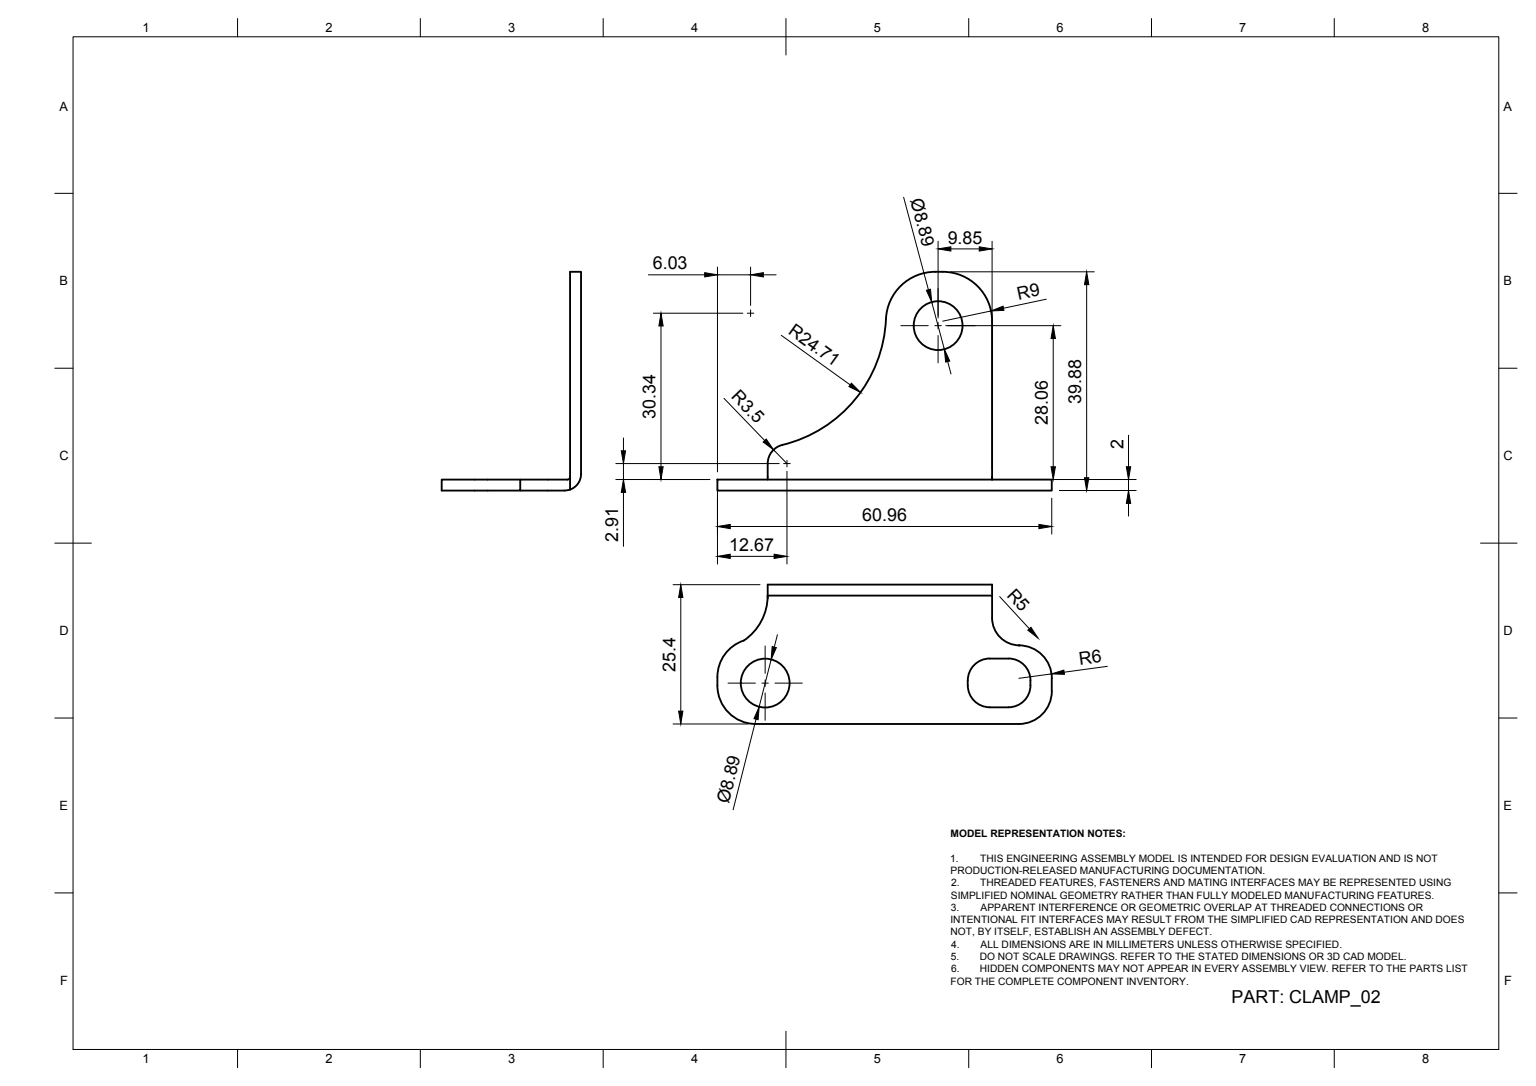
ISO-10303-21;
HEADER;
/* Generated by software containing ST-Developer
 * from STEP Tools, Inc. (www.steptools.com) 
 */

FILE_DESCRIPTION(
/* description */ (''),
/* implementation_level */ '2;1');

FILE_NAME(
/* name */ 'Clamp_02.step',
/* time_stamp */ '2026-10-04T16:49:01-07:00',
/* author */ (''),
/* organization */ (''),
/* preprocessor_version */ 'ST-DEVELOPER v20.2',
/* originating_system */ 'Autodesk Translation Framework v15.15.0.0',
/* authorisation */ '');

FILE_SCHEMA (('AUTOMOTIVE_DESIGN { 1 0 10303 214 3 1 1 }'));
ENDSEC;

DATA;
#10=MECHANICAL_DESIGN_GEOMETRIC_PRESENTATION_REPRESENTATION('',(#86),#51553);
#70=SHAPE_REPRESENTATION_RELATIONSHIP('SRR','None',#51591,#78);
#78=ADVANCED_BREP_SHAPE_REPRESENTATION('',(#95),#51551);
#86=STYLED_ITEM('',(#51634),#95);
#95=MANIFOLD_SOLID_BREP('Body1',#4265);
#110=FACE_BOUND('',#538,.T.);
#111=FACE_BOUND('',#541,.T.);
#112=FACE_BOUND('',#570,.T.);
#113=FACE_BOUND('',#571,.T.);
#114=FACE_BOUND('',#573,.T.);
#115=FACE_BOUND('',#574,.T.);
#159=PLANE('',#4564);
#160=PLANE('',#4566);
#161=PLANE('',#4572);
#162=PLANE('',#4573);
#163=PLANE('',#4584);
#164=PLANE('',#4587);
#165=PLANE('',#4591);
#166=PLANE('',#4595);
#167=PLANE('',#4599);
#168=PLANE('',#4603);
#169=PLANE('',#4616);
#170=PLANE('',#4620);
#171=PLANE('',#4624);
#172=PLANE('',#4628);
#173=PLANE('',#4629);
#174=PLANE('',#4630);
#328=FACE_OUTER_BOUND('',#535,.T.);
#329=FACE_OUTER_BOUND('',#536,.T.);
#330=FACE_OUTER_BOUND('',#537,.T.);
#331=FACE_OUTER_BOUND('',#539,.T.);
#332=FACE_OUTER_BOUND('',#540,.T.);
#333=FACE_OUTER_BOUND('',#542,.T.);
#334=FACE_OUTER_BOUND('',#543,.T.);
#335=FACE_OUTER_BOUND('',#544,.T.);
#336=FACE_OUTER_BOUND('',#545,.T.);
#337=FACE_OUTER_BOUND('',#546,.T.);
#338=FACE_OUTER_BOUND('',#547,.T.);
#339=FACE_OUTER_BOUND('',#548,.T.);
#340=FACE_OUTER_BOUND('',#549,.T.);
#341=FACE_OUTER_BOUND('',#550,.T.);
#342=FACE_OUTER_BOUND('',#551,.T.);
#343=FACE_OUTER_BOUND('',#552,.T.);
#344=FACE_OUTER_BOUND('',#553,.T.);
#345=FACE_OUTER_BOUND('',#554,.T.);
#346=FACE_OUTER_BOUND('',#555,.T.);
#347=FACE_OUTER_BOUND('',#556,.T.);
#348=FACE_OUTER_BOUND('',#557,.T.);
#349=FACE_OUTER_BOUND('',#558,.T.);
#350=FACE_OUTER_BOUND('',#559,.T.);
#351=FACE_OUTER_BOUND('',#560,.T.);
#352=FACE_OUTER_BOUND('',#561,.T.);
#353=FACE_OUTER_BOUND('',#562,.T.);
#354=FACE_OUTER_BOUND('',#563,.T.);
#355=FACE_OUTER_BOUND('',#564,.T.);
#356=FACE_OUTER_BOUND('',#565,.T.);
#357=FACE_OUTER_BOUND('',#566,.T.);
#358=FACE_OUTER_BOUND('',#567,.T.);
#359=FACE_OUTER_BOUND('',#568,.T.);
#360=FACE_OUTER_BOUND('',#569,.T.);
#361=FACE_OUTER_BOUND('',#572,.T.);
#535=EDGE_LOOP('',(#3703,#3704,#3705,#3706,#3707,#3708,#3709));
#536=EDGE_LOOP('',(#3710,#3711,#3712,#3713,#3714,#3715));
#537=EDGE_LOOP('',(#3716,#3717,#3718,#3719,#3720,#3721,#3722,#3723,#3724,
#3725));
#538=EDGE_LOOP('',(#3726));
#539=EDGE_LOOP('',(#3727,#3728,#3729,#3730));
#540=EDGE_LOOP('',(#3731,#3732,#3733,#3734,#3735,#3736,#3737,#3738));
#541=EDGE_LOOP('',(#3739));
#542=EDGE_LOOP('',(#3740,#3741,#3742,#3743));
#543=EDGE_LOOP('',(#3744,#3745,#3746,#3747));
#544=EDGE_LOOP('',(#3748,#3749,#3750,#3751));
#545=EDGE_LOOP('',(#3752,#3753,#3754,#3755));
#546=EDGE_LOOP('',(#3756,#3757,#3758,#3759));
#547=EDGE_LOOP('',(#3760,#3761,#3762,#3763));
#548=EDGE_LOOP('',(#3764,#3765,#3766,#3767));
#549=EDGE_LOOP('',(#3768,#3769,#3770,#3771,#3772,#3773,#3774));
#550=EDGE_LOOP('',(#3775,#3776,#3777,#3778));
#551=EDGE_LOOP('',(#3779,#3780,#3781,#3782));
#552=EDGE_LOOP('',(#3783,#3784,#3785,#3786));
#553=EDGE_LOOP('',(#3787,#3788,#3789,#3790));
#554=EDGE_LOOP('',(#3791,#3792,#3793,#3794));
#555=EDGE_LOOP('',(#3795,#3796,#3797,#3798));
#556=EDGE_LOOP('',(#3799,#3800,#3801,#3802));
#557=EDGE_LOOP('',(#3803,#3804,#3805,#3806));
#558=EDGE_LOOP('',(#3807,#3808,#3809,#3810));
#559=EDGE_LOOP('',(#3811,#3812,#3813,#3814));
#560=EDGE_LOOP('',(#3815,#3816,#3817,#3818,#3819));
#561=EDGE_LOOP('',(#3820,#3821,#3822,#3823));
#562=EDGE_LOOP('',(#3824,#3825,#3826,#3827));
#563=EDGE_LOOP('',(#3828,#3829,#3830,#3831));
#564=EDGE_LOOP('',(#3832,#3833,#3834,#3835));
#565=EDGE_LOOP('',(#3836,#3837,#3838,#3839));
#566=EDGE_LOOP('',(#3840,#3841,#3842,#3843));
#567=EDGE_LOOP('',(#3844,#3845,#3846,#3847));
#568=EDGE_LOOP('',(#3848,#3849,#3850,#3851));
#569=EDGE_LOOP('',(#3852,#3853,#3854,#3855,#3856,#3857,#3858,#3859,#3860,
#3861,#3862,#3863,#3864));
#570=EDGE_LOOP('',(#3865,#3866,#3867,#3868,#3869,#3870,#3871,#3872));
#571=EDGE_LOOP('',(#3873));
#572=EDGE_LOOP('',(#3874,#3875,#3876,#3877,#3878,#3879,#3880,#3881,#3882,
#3883,#3884,#3885));
#573=EDGE_LOOP('',(#3886,#3887,#3888,#3889,#3890,#3891,#3892,#3893));
#574=EDGE_LOOP('',(#3894));
#657=CIRCLE('',#4561,3.);
#658=CIRCLE('',#4562,3.);
#659=CIRCLE('',#4563,3.);
#660=CIRCLE('',#4565,0.5);
#661=CIRCLE('',#4567,9.);
#662=CIRCLE('',#4568,9.);
#663=CIRCLE('',#4569,24.7141941620437);
#664=CIRCLE('',#4570,3.5);
#665=CIRCLE('',#4571,4.445);
#666=CIRCLE('',#4574,3.5);
#667=CIRCLE('',#4575,24.7141941620437);
#668=CIRCLE('',#4576,9.);
#669=CIRCLE('',#4577,9.);
#670=CIRCLE('',#4578,4.445);
#671=CIRCLE('',#4580,0.5);
#672=CIRCLE('',#4589,4.445);
#673=CIRCLE('',#4590,4.445);
#674=CIRCLE('',#4593,3.99999999999999);
#675=CIRCLE('',#4594,3.99999999999999);
#676=CIRCLE('',#4597,4.00000000000001);
#677=CIRCLE('',#4598,4.00000000000001);
#678=CIRCLE('',#4601,4.00000000000001);
#679=CIRCLE('',#4602,4.00000000000001);
#680=CIRCLE('',#4605,4.00000000000001);
#681=CIRCLE('',#4606,4.00000000000001);
#682=CIRCLE('',#4608,6.99999999999999);
#683=CIRCLE('',#4609,6.99999999999999);
#684=CIRCLE('',#4611,9.9094315895918);
#685=CIRCLE('',#4612,9.9094315895918);
#686=CIRCLE('',#4614,5.);
#687=CIRCLE('',#4615,5.);
#688=CIRCLE('',#4618,5.99999999999999);
#689=CIRCLE('',#4619,5.99999999999999);
#690=CIRCLE('',#4622,5.99999999999999);
#691=CIRCLE('',#4623,5.99999999999999);
#692=CIRCLE('',#4626,7.);
#693=CIRCLE('',#4627,7.);
#872=LINE('',#51257,#1100);
#873=LINE('',#51261,#1101);
#874=LINE('',#51265,#1102);
#875=LINE('',#51272,#1103);
#876=LINE('',#51276,#1104);
#877=LINE('',#51278,#1105);
#878=LINE('',#51279,#1106);
#879=LINE('',#51282,#1107);
#880=LINE('',#51286,#1108);
#881=LINE('',#51294,#1109);
#882=LINE('',#51295,#1110);
#883=LINE('',#51300,#1111);
#884=LINE('',#51301,#1112);
#885=LINE('',#51304,#1113);
#886=LINE('',#51312,#1114);
#887=LINE('',#51319,#1115);
#888=LINE('',#51321,#1116);
#889=LINE('',#51322,#1117);
#890=LINE('',#51324,#1118);
#891=LINE('',#51326,#1119);
#892=LINE('',#51328,#1120);
#893=LINE('',#51331,#1121);
#894=LINE('',#51334,#1122);
#895=LINE('',#51335,#1123);
#896=LINE('',#51340,#1124);
#897=LINE('',#51345,#1125);
#898=LINE('',#51347,#1126);
#899=LINE('',#51349,#1127);
#900=LINE('',#51350,#1128);
#901=LINE('',#51356,#1129);
#902=LINE('',#51359,#1130);
#903=LINE('',#51361,#1131);
#904=LINE('',#51362,#1132);
#905=LINE('',#51368,#1133);
#906=LINE('',#51371,#1134);
#907=LINE('',#51373,#1135);
#908=LINE('',#51374,#1136);
#909=LINE('',#51380,#1137);
#910=LINE('',#51383,#1138);
#911=LINE('',#51385,#1139);
#912=LINE('',#51386,#1140);
#913=LINE('',#51395,#1141);
#914=LINE('',#51398,#1142);
#915=LINE('',#51407,#1143);
#916=LINE('',#51410,#1144);
#917=LINE('',#51412,#1145);
#918=LINE('',#51413,#1146);
#919=LINE('',#51419,#1147);
#920=LINE('',#51422,#1148);
#921=LINE('',#51424,#1149);
#922=LINE('',#51425,#1150);
#923=LINE('',#51431,#1151);
#924=LINE('',#51434,#1152);
#925=LINE('',#51436,#1153);
#926=LINE('',#51437,#1154);
#927=LINE('',#51443,#1155);
#928=LINE('',#51445,#1156);
#929=LINE('',#51446,#1157);
#1100=VECTOR('',#5242,10.);
#1101=VECTOR('',#5245,10.);
#1102=VECTOR('',#5248,10.);
#1103=VECTOR('',#5251,10.);
#1104=VECTOR('',#5254,10.);
#1105=VECTOR('',#5255,10.);
#1106=VECTOR('',#5256,10.);
#1107=VECTOR('',#5259,10.);
#1108=VECTOR('',#5262,10.);
#1109=VECTOR('',#5269,10.);
#1110=VECTOR('',#5270,10.);
#1111=VECTOR('',#5275,10.);
#1112=VECTOR('',#5276,10.);
#1113=VECTOR('',#5279,10.);
#1114=VECTOR('',#5286,10.);
#1115=VECTOR('',#5295,10.);
#1116=VECTOR('',#5298,10.);
#1117=VECTOR('',#5299,10.);
#1118=VECTOR('',#5302,9.);
#1119=VECTOR('',#5305,10.);
#1120=VECTOR('',#5308,9.);
#1121=VECTOR('',#5313,4.445);
#1122=VECTOR('',#5316,10.);
#1123=VECTOR('',#5317,10.);
#1124=VECTOR('',#5322,4.445);
#1125=VECTOR('',#5327,10.);
#1126=VECTOR('',#5328,10.);
#1127=VECTOR('',#5329,10.);
#1128=VECTOR('',#5330,10.);
#1129=VECTOR('',#5337,10.);
#1130=VECTOR('',#5340,10.);
#1131=VECTOR('',#5341,10.);
#1132=VECTOR('',#5342,10.);
#1133=VECTOR('',#5349,10.);
#1134=VECTOR('',#5352,10.);
#1135=VECTOR('',#5353,10.);
#1136=VECTOR('',#5354,10.);
#1137=VECTOR('',#5361,10.);
#1138=VECTOR('',#5364,10.);
#1139=VECTOR('',#5365,10.);
#1140=VECTOR('',#5366,10.);
#1141=VECTOR('',#5377,10.);
#1142=VECTOR('',#5380,10.);
#1143=VECTOR('',#5393,10.);
#1144=VECTOR('',#5396,10.);
#1145=VECTOR('',#5397,10.);
#1146=VECTOR('',#5398,10.);
#1147=VECTOR('',#5405,10.);
#1148=VECTOR('',#5408,10.);
#1149=VECTOR('',#5409,10.);
#1150=VECTOR('',#5410,10.);
#1151=VECTOR('',#5417,10.);
#1152=VECTOR('',#5420,10.);
#1153=VECTOR('',#5421,10.);
#1154=VECTOR('',#5422,10.);
#1155=VECTOR('',#5429,10.);
#1156=VECTOR('',#5432,10.);
#1157=VECTOR('',#5433,10.);
#1479=B_SPLINE_CURVE_WITH_KNOTS('',3,(#51266,#51267,#51268,#51269),
 .UNSPECIFIED.,.F.,.F.,(4,4),(-0.453207372117249,-0.354837975954888),
 .UNSPECIFIED.);
#1884=VERTEX_POINT('',#51253);
#1885=VERTEX_POINT('',#51254);
#1886=VERTEX_POINT('',#51256);
#1887=VERTEX_POINT('',#51258);
#1888=VERTEX_POINT('',#51260);
#1889=VERTEX_POINT('',#51262);
#1890=VERTEX_POINT('',#51264);
#1891=VERTEX_POINT('',#51271);
#1892=VERTEX_POINT('',#51273);
#1893=VERTEX_POINT('',#51275);
#1894=VERTEX_POINT('',#51277);
#1895=VERTEX_POINT('',#51281);
#1896=VERTEX_POINT('',#51283);
#1897=VERTEX_POINT('',#51285);
#1898=VERTEX_POINT('',#51287);
#1899=VERTEX_POINT('',#51289);
#1900=VERTEX_POINT('',#51291);
#1901=VERTEX_POINT('',#51293);
#1902=VERTEX_POINT('',#51296);
#1903=VERTEX_POINT('',#51299);
#1904=VERTEX_POINT('',#51303);
#1905=VERTEX_POINT('',#51305);
#1906=VERTEX_POINT('',#51307);
#1907=VERTEX_POINT('',#51309);
#1908=VERTEX_POINT('',#51311);
#1909=VERTEX_POINT('',#51314);
#1910=VERTEX_POINT('',#51317);
#1911=VERTEX_POINT('',#51333);
#1912=VERTEX_POINT('',#51337);
#1913=VERTEX_POINT('',#51339);
#1914=VERTEX_POINT('',#51343);
#1915=VERTEX_POINT('',#51344);
#1916=VERTEX_POINT('',#51346);
#1917=VERTEX_POINT('',#51348);
#1918=VERTEX_POINT('',#51352);
#1919=VERTEX_POINT('',#51354);
#1920=VERTEX_POINT('',#51358);
#1921=VERTEX_POINT('',#51360);
#1922=VERTEX_POINT('',#51364);
#1923=VERTEX_POINT('',#51366);
#1924=VERTEX_POINT('',#51370);
#1925=VERTEX_POINT('',#51372);
#1926=VERTEX_POINT('',#51376);
#1927=VERTEX_POINT('',#51378);
#1928=VERTEX_POINT('',#51382);
#1929=VERTEX_POINT('',#51384);
#1930=VERTEX_POINT('',#51391);
#1931=VERTEX_POINT('',#51392);
#1932=VERTEX_POINT('',#51394);
#1933=VERTEX_POINT('',#51396);
#1934=VERTEX_POINT('',#51403);
#1935=VERTEX_POINT('',#51405);
#1936=VERTEX_POINT('',#51409);
#1937=VERTEX_POINT('',#51411);
#1938=VERTEX_POINT('',#51415);
#1939=VERTEX_POINT('',#51417);
#1940=VERTEX_POINT('',#51421);
#1941=VERTEX_POINT('',#51423);
#1942=VERTEX_POINT('',#51427);
#1943=VERTEX_POINT('',#51429);
#1944=VERTEX_POINT('',#51433);
#1945=VERTEX_POINT('',#51435);
#1946=VERTEX_POINT('',#51439);
#1947=VERTEX_POINT('',#51441);
#2505=EDGE_CURVE('',#1884,#1885,#657,.T.);
#2506=EDGE_CURVE('',#1885,#1886,#872,.T.);
#2507=EDGE_CURVE('',#1886,#1887,#658,.T.);
#2508=EDGE_CURVE('',#1887,#1888,#873,.T.);
#2509=EDGE_CURVE('',#1888,#1889,#659,.T.);
#2510=EDGE_CURVE('',#1889,#1890,#874,.T.);
#2511=EDGE_CURVE('',#1890,#1884,#1479,.T.);
#2512=EDGE_CURVE('',#1888,#1891,#875,.T.);
#2513=EDGE_CURVE('',#1892,#1891,#660,.T.);
#2514=EDGE_CURVE('',#1893,#1892,#876,.T.);
#2515=EDGE_CURVE('',#1894,#1893,#877,.T.);
#2516=EDGE_CURVE('',#1894,#1889,#878,.T.);
#2517=EDGE_CURVE('',#1887,#1895,#879,.F.);
#2518=EDGE_CURVE('',#1896,#1895,#661,.T.);
#2519=EDGE_CURVE('',#1897,#1896,#880,.T.);
#2520=EDGE_CURVE('',#1898,#1897,#662,.T.);
#2521=EDGE_CURVE('',#1898,#1899,#663,.T.);
#2522=EDGE_CURVE('',#1900,#1899,#664,.T.);
#2523=EDGE_CURVE('',#1901,#1900,#881,.T.);
#2524=EDGE_CURVE('',#1891,#1901,#882,.T.);
#2525=EDGE_CURVE('',#1902,#1902,#665,.T.);
#2526=EDGE_CURVE('',#1886,#1903,#883,.T.);
#2527=EDGE_CURVE('',#1895,#1903,#884,.T.);
#2528=EDGE_CURVE('',#1885,#1904,#885,.F.);
#2529=EDGE_CURVE('',#1905,#1904,#666,.T.);
#2530=EDGE_CURVE('',#1905,#1906,#667,.T.);
#2531=EDGE_CURVE('',#1907,#1906,#668,.T.);
#2532=EDGE_CURVE('',#1908,#1907,#886,.T.);
#2533=EDGE_CURVE('',#1903,#1908,#669,.T.);
#2534=EDGE_CURVE('',#1909,#1909,#670,.T.);
#2535=EDGE_CURVE('',#1910,#1901,#671,.F.);
#2536=EDGE_CURVE('',#1910,#1892,#887,.T.);
#2537=EDGE_CURVE('',#1904,#1900,#888,.T.);
#2538=EDGE_CURVE('',#1899,#1905,#889,.T.);
#2539=EDGE_CURVE('',#1906,#1898,#890,.T.);
#2540=EDGE_CURVE('',#1908,#1896,#891,.T.);
#2541=EDGE_CURVE('',#1897,#1907,#892,.T.);
#2542=EDGE_CURVE('',#1902,#1909,#893,.T.);
#2543=EDGE_CURVE('',#1884,#1911,#894,.T.);
#2544=EDGE_CURVE('',#1910,#1911,#895,.T.);
#2545=EDGE_CURVE('',#1912,#1912,#672,.T.);
#2546=EDGE_CURVE('',#1912,#1913,#896,.T.);
#2547=EDGE_CURVE('',#1913,#1913,#673,.T.);
#2548=EDGE_CURVE('',#1914,#1915,#897,.T.);
#2549=EDGE_CURVE('',#1915,#1916,#898,.T.);
#2550=EDGE_CURVE('',#1917,#1916,#899,.T.);
#2551=EDGE_CURVE('',#1914,#1917,#900,.T.);
#2552=EDGE_CURVE('',#1918,#1914,#674,.T.);
#2553=EDGE_CURVE('',#1919,#1917,#675,.T.);
#2554=EDGE_CURVE('',#1918,#1919,#901,.T.);
#2555=EDGE_CURVE('',#1920,#1918,#902,.T.);
#2556=EDGE_CURVE('',#1921,#1919,#903,.T.);
#2557=EDGE_CURVE('',#1920,#1921,#904,.T.);
#2558=EDGE_CURVE('',#1922,#1920,#676,.T.);
#2559=EDGE_CURVE('',#1923,#1921,#677,.T.);
#2560=EDGE_CURVE('',#1922,#1923,#905,.T.);
#2561=EDGE_CURVE('',#1924,#1922,#906,.T.);
#2562=EDGE_CURVE('',#1925,#1923,#907,.T.);
#2563=EDGE_CURVE('',#1924,#1925,#908,.T.);
#2564=EDGE_CURVE('',#1926,#1924,#678,.T.);
#2565=EDGE_CURVE('',#1927,#1925,#679,.T.);
#2566=EDGE_CURVE('',#1926,#1927,#909,.T.);
#2567=EDGE_CURVE('',#1928,#1926,#910,.T.);
#2568=EDGE_CURVE('',#1929,#1927,#911,.T.);
#2569=EDGE_CURVE('',#1928,#1929,#912,.T.);
#2570=EDGE_CURVE('',#1915,#1928,#680,.T.);
#2571=EDGE_CURVE('',#1916,#1929,#681,.T.);
#2572=EDGE_CURVE('',#1930,#1931,#682,.T.);
#2573=EDGE_CURVE('',#1931,#1932,#913,.T.);
#2574=EDGE_CURVE('',#1933,#1932,#683,.T.);
#2575=EDGE_CURVE('',#1930,#1933,#914,.T.);
#2576=EDGE_CURVE('',#1930,#1890,#684,.T.);
#2577=EDGE_CURVE('',#1911,#1933,#685,.T.);
#2578=EDGE_CURVE('',#1894,#1934,#686,.T.);
#2579=EDGE_CURVE('',#1935,#1893,#687,.T.);
#2580=EDGE_CURVE('',#1934,#1935,#915,.T.);
#2581=EDGE_CURVE('',#1936,#1934,#916,.T.);
#2582=EDGE_CURVE('',#1937,#1935,#917,.T.);
#2583=EDGE_CURVE('',#1936,#1937,#918,.T.);
#2584=EDGE_CURVE('',#1938,#1936,#688,.T.);
#2585=EDGE_CURVE('',#1939,#1937,#689,.T.);
#2586=EDGE_CURVE('',#1938,#1939,#919,.T.);
#2587=EDGE_CURVE('',#1940,#1938,#920,.T.);
#2588=EDGE_CURVE('',#1941,#1939,#921,.T.);
#2589=EDGE_CURVE('',#1940,#1941,#922,.T.);
#2590=EDGE_CURVE('',#1942,#1940,#690,.T.);
#2591=EDGE_CURVE('',#1943,#1941,#691,.T.);
#2592=EDGE_CURVE('',#1942,#1943,#923,.T.);
#2593=EDGE_CURVE('',#1944,#1942,#924,.T.);
#2594=EDGE_CURVE('',#1945,#1943,#925,.T.);
#2595=EDGE_CURVE('',#1944,#1945,#926,.T.);
#2596=EDGE_CURVE('',#1946,#1944,#692,.T.);
#2597=EDGE_CURVE('',#1947,#1945,#693,.T.);
#2598=EDGE_CURVE('',#1946,#1947,#927,.T.);
#2599=EDGE_CURVE('',#1931,#1946,#928,.T.);
#2600=EDGE_CURVE('',#1932,#1947,#929,.T.);
#3703=ORIENTED_EDGE('',*,*,#2505,.T.);
#3704=ORIENTED_EDGE('',*,*,#2506,.T.);
#3705=ORIENTED_EDGE('',*,*,#2507,.T.);
#3706=ORIENTED_EDGE('',*,*,#2508,.T.);
#3707=ORIENTED_EDGE('',*,*,#2509,.T.);
#3708=ORIENTED_EDGE('',*,*,#2510,.T.);
#3709=ORIENTED_EDGE('',*,*,#2511,.T.);
#3710=ORIENTED_EDGE('',*,*,#2509,.F.);
#3711=ORIENTED_EDGE('',*,*,#2512,.T.);
#3712=ORIENTED_EDGE('',*,*,#2513,.F.);
#3713=ORIENTED_EDGE('',*,*,#2514,.F.);
#3714=ORIENTED_EDGE('',*,*,#2515,.F.);
#3715=ORIENTED_EDGE('',*,*,#2516,.T.);
#3716=ORIENTED_EDGE('',*,*,#2508,.F.);
#3717=ORIENTED_EDGE('',*,*,#2517,.T.);
#3718=ORIENTED_EDGE('',*,*,#2518,.F.);
#3719=ORIENTED_EDGE('',*,*,#2519,.F.);
#3720=ORIENTED_EDGE('',*,*,#2520,.F.);
#3721=ORIENTED_EDGE('',*,*,#2521,.T.);
#3722=ORIENTED_EDGE('',*,*,#2522,.F.);
#3723=ORIENTED_EDGE('',*,*,#2523,.F.);
#3724=ORIENTED_EDGE('',*,*,#2524,.F.);
#3725=ORIENTED_EDGE('',*,*,#2512,.F.);
#3726=ORIENTED_EDGE('',*,*,#2525,.T.);
#3727=ORIENTED_EDGE('',*,*,#2507,.F.);
#3728=ORIENTED_EDGE('',*,*,#2526,.T.);
#3729=ORIENTED_EDGE('',*,*,#2527,.F.);
#3730=ORIENTED_EDGE('',*,*,#2517,.F.);
#3731=ORIENTED_EDGE('',*,*,#2506,.F.);
#3732=ORIENTED_EDGE('',*,*,#2528,.T.);
#3733=ORIENTED_EDGE('',*,*,#2529,.F.);
#3734=ORIENTED_EDGE('',*,*,#2530,.T.);
#3735=ORIENTED_EDGE('',*,*,#2531,.F.);
#3736=ORIENTED_EDGE('',*,*,#2532,.F.);
#3737=ORIENTED_EDGE('',*,*,#2533,.F.);
#3738=ORIENTED_EDGE('',*,*,#2526,.F.);
#3739=ORIENTED_EDGE('',*,*,#2534,.T.);
#3740=ORIENTED_EDGE('',*,*,#2535,.F.);
#3741=ORIENTED_EDGE('',*,*,#2536,.T.);
#3742=ORIENTED_EDGE('',*,*,#2513,.T.);
#3743=ORIENTED_EDGE('',*,*,#2524,.T.);
#3744=ORIENTED_EDGE('',*,*,#2529,.T.);
#3745=ORIENTED_EDGE('',*,*,#2537,.T.);
#3746=ORIENTED_EDGE('',*,*,#2522,.T.);
#3747=ORIENTED_EDGE('',*,*,#2538,.T.);
#3748=ORIENTED_EDGE('',*,*,#2538,.F.);
#3749=ORIENTED_EDGE('',*,*,#2521,.F.);
#3750=ORIENTED_EDGE('',*,*,#2539,.F.);
#3751=ORIENTED_EDGE('',*,*,#2530,.F.);
#3752=ORIENTED_EDGE('',*,*,#2533,.T.);
#3753=ORIENTED_EDGE('',*,*,#2540,.T.);
#3754=ORIENTED_EDGE('',*,*,#2518,.T.);
#3755=ORIENTED_EDGE('',*,*,#2527,.T.);
#3756=ORIENTED_EDGE('',*,*,#2540,.F.);
#3757=ORIENTED_EDGE('',*,*,#2532,.T.);
#3758=ORIENTED_EDGE('',*,*,#2541,.F.);
#3759=ORIENTED_EDGE('',*,*,#2519,.T.);
#3760=ORIENTED_EDGE('',*,*,#2531,.T.);
#3761=ORIENTED_EDGE('',*,*,#2539,.T.);
#3762=ORIENTED_EDGE('',*,*,#2520,.T.);
#3763=ORIENTED_EDGE('',*,*,#2541,.T.);
#3764=ORIENTED_EDGE('',*,*,#2525,.F.);
#3765=ORIENTED_EDGE('',*,*,#2542,.T.);
#3766=ORIENTED_EDGE('',*,*,#2534,.F.);
#3767=ORIENTED_EDGE('',*,*,#2542,.F.);
#3768=ORIENTED_EDGE('',*,*,#2505,.F.);
#3769=ORIENTED_EDGE('',*,*,#2543,.T.);
#3770=ORIENTED_EDGE('',*,*,#2544,.F.);
#3771=ORIENTED_EDGE('',*,*,#2535,.T.);
#3772=ORIENTED_EDGE('',*,*,#2523,.T.);
#3773=ORIENTED_EDGE('',*,*,#2537,.F.);
#3774=ORIENTED_EDGE('',*,*,#2528,.F.);
#3775=ORIENTED_EDGE('',*,*,#2545,.T.);
#3776=ORIENTED_EDGE('',*,*,#2546,.T.);
#3777=ORIENTED_EDGE('',*,*,#2547,.F.);
#3778=ORIENTED_EDGE('',*,*,#2546,.F.);
#3779=ORIENTED_EDGE('',*,*,#2548,.T.);
#3780=ORIENTED_EDGE('',*,*,#2549,.T.);
#3781=ORIENTED_EDGE('',*,*,#2550,.F.);
#3782=ORIENTED_EDGE('',*,*,#2551,.F.);
#3783=ORIENTED_EDGE('',*,*,#2552,.T.);
#3784=ORIENTED_EDGE('',*,*,#2551,.T.);
#3785=ORIENTED_EDGE('',*,*,#2553,.F.);
#3786=ORIENTED_EDGE('',*,*,#2554,.F.);
#3787=ORIENTED_EDGE('',*,*,#2555,.T.);
#3788=ORIENTED_EDGE('',*,*,#2554,.T.);
#3789=ORIENTED_EDGE('',*,*,#2556,.F.);
#3790=ORIENTED_EDGE('',*,*,#2557,.F.);
#3791=ORIENTED_EDGE('',*,*,#2558,.T.);
#3792=ORIENTED_EDGE('',*,*,#2557,.T.);
#3793=ORIENTED_EDGE('',*,*,#2559,.F.);
#3794=ORIENTED_EDGE('',*,*,#2560,.F.);
#3795=ORIENTED_EDGE('',*,*,#2561,.T.);
#3796=ORIENTED_EDGE('',*,*,#2560,.T.);
#3797=ORIENTED_EDGE('',*,*,#2562,.F.);
#3798=ORIENTED_EDGE('',*,*,#2563,.F.);
#3799=ORIENTED_EDGE('',*,*,#2564,.T.);
#3800=ORIENTED_EDGE('',*,*,#2563,.T.);
#3801=ORIENTED_EDGE('',*,*,#2565,.F.);
#3802=ORIENTED_EDGE('',*,*,#2566,.F.);
#3803=ORIENTED_EDGE('',*,*,#2567,.T.);
#3804=ORIENTED_EDGE('',*,*,#2566,.T.);
#3805=ORIENTED_EDGE('',*,*,#2568,.F.);
#3806=ORIENTED_EDGE('',*,*,#2569,.F.);
#3807=ORIENTED_EDGE('',*,*,#2570,.T.);
#3808=ORIENTED_EDGE('',*,*,#2569,.T.);
#3809=ORIENTED_EDGE('',*,*,#2571,.F.);
#3810=ORIENTED_EDGE('',*,*,#2549,.F.);
#3811=ORIENTED_EDGE('',*,*,#2572,.T.);
#3812=ORIENTED_EDGE('',*,*,#2573,.T.);
#3813=ORIENTED_EDGE('',*,*,#2574,.F.);
#3814=ORIENTED_EDGE('',*,*,#2575,.F.);
#3815=ORIENTED_EDGE('',*,*,#2511,.F.);
#3816=ORIENTED_EDGE('',*,*,#2576,.F.);
#3817=ORIENTED_EDGE('',*,*,#2575,.T.);
#3818=ORIENTED_EDGE('',*,*,#2577,.F.);
#3819=ORIENTED_EDGE('',*,*,#2543,.F.);
#3820=ORIENTED_EDGE('',*,*,#2578,.F.);
#3821=ORIENTED_EDGE('',*,*,#2515,.T.);
#3822=ORIENTED_EDGE('',*,*,#2579,.F.);
#3823=ORIENTED_EDGE('',*,*,#2580,.F.);
#3824=ORIENTED_EDGE('',*,*,#2581,.T.);
#3825=ORIENTED_EDGE('',*,*,#2580,.T.);
#3826=ORIENTED_EDGE('',*,*,#2582,.F.);
#3827=ORIENTED_EDGE('',*,*,#2583,.F.);
#3828=ORIENTED_EDGE('',*,*,#2584,.T.);
#3829=ORIENTED_EDGE('',*,*,#2583,.T.);
#3830=ORIENTED_EDGE('',*,*,#2585,.F.);
#3831=ORIENTED_EDGE('',*,*,#2586,.F.);
#3832=ORIENTED_EDGE('',*,*,#2587,.T.);
#3833=ORIENTED_EDGE('',*,*,#2586,.T.);
#3834=ORIENTED_EDGE('',*,*,#2588,.F.);
#3835=ORIENTED_EDGE('',*,*,#2589,.F.);
#3836=ORIENTED_EDGE('',*,*,#2590,.T.);
#3837=ORIENTED_EDGE('',*,*,#2589,.T.);
#3838=ORIENTED_EDGE('',*,*,#2591,.F.);
#3839=ORIENTED_EDGE('',*,*,#2592,.F.);
#3840=ORIENTED_EDGE('',*,*,#2593,.T.);
#3841=ORIENTED_EDGE('',*,*,#2592,.T.);
#3842=ORIENTED_EDGE('',*,*,#2594,.F.);
#3843=ORIENTED_EDGE('',*,*,#2595,.F.);
#3844=ORIENTED_EDGE('',*,*,#2596,.T.);
#3845=ORIENTED_EDGE('',*,*,#2595,.T.);
#3846=ORIENTED_EDGE('',*,*,#2597,.F.);
#3847=ORIENTED_EDGE('',*,*,#2598,.F.);
#3848=ORIENTED_EDGE('',*,*,#2599,.T.);
#3849=ORIENTED_EDGE('',*,*,#2598,.T.);
#3850=ORIENTED_EDGE('',*,*,#2600,.F.);
#3851=ORIENTED_EDGE('',*,*,#2573,.F.);
#3852=ORIENTED_EDGE('',*,*,#2577,.T.);
#3853=ORIENTED_EDGE('',*,*,#2574,.T.);
#3854=ORIENTED_EDGE('',*,*,#2600,.T.);
#3855=ORIENTED_EDGE('',*,*,#2597,.T.);
#3856=ORIENTED_EDGE('',*,*,#2594,.T.);
#3857=ORIENTED_EDGE('',*,*,#2591,.T.);
#3858=ORIENTED_EDGE('',*,*,#2588,.T.);
#3859=ORIENTED_EDGE('',*,*,#2585,.T.);
#3860=ORIENTED_EDGE('',*,*,#2582,.T.);
#3861=ORIENTED_EDGE('',*,*,#2579,.T.);
#3862=ORIENTED_EDGE('',*,*,#2514,.T.);
#3863=ORIENTED_EDGE('',*,*,#2536,.F.);
#3864=ORIENTED_EDGE('',*,*,#2544,.T.);
#3865=ORIENTED_EDGE('',*,*,#2571,.T.);
#3866=ORIENTED_EDGE('',*,*,#2568,.T.);
#3867=ORIENTED_EDGE('',*,*,#2565,.T.);
#3868=ORIENTED_EDGE('',*,*,#2562,.T.);
#3869=ORIENTED_EDGE('',*,*,#2559,.T.);
#3870=ORIENTED_EDGE('',*,*,#2556,.T.);
#3871=ORIENTED_EDGE('',*,*,#2553,.T.);
#3872=ORIENTED_EDGE('',*,*,#2550,.T.);
#3873=ORIENTED_EDGE('',*,*,#2547,.T.);
#3874=ORIENTED_EDGE('',*,*,#2510,.F.);
#3875=ORIENTED_EDGE('',*,*,#2516,.F.);
#3876=ORIENTED_EDGE('',*,*,#2578,.T.);
#3877=ORIENTED_EDGE('',*,*,#2581,.F.);
#3878=ORIENTED_EDGE('',*,*,#2584,.F.);
#3879=ORIENTED_EDGE('',*,*,#2587,.F.);
#3880=ORIENTED_EDGE('',*,*,#2590,.F.);
#3881=ORIENTED_EDGE('',*,*,#2593,.F.);
#3882=ORIENTED_EDGE('',*,*,#2596,.F.);
#3883=ORIENTED_EDGE('',*,*,#2599,.F.);
#3884=ORIENTED_EDGE('',*,*,#2572,.F.);
#3885=ORIENTED_EDGE('',*,*,#2576,.T.);
#3886=ORIENTED_EDGE('',*,*,#2570,.F.);
#3887=ORIENTED_EDGE('',*,*,#2548,.F.);
#3888=ORIENTED_EDGE('',*,*,#2552,.F.);
#3889=ORIENTED_EDGE('',*,*,#2555,.F.);
#3890=ORIENTED_EDGE('',*,*,#2558,.F.);
#3891=ORIENTED_EDGE('',*,*,#2561,.F.);
#3892=ORIENTED_EDGE('',*,*,#2564,.F.);
#3893=ORIENTED_EDGE('',*,*,#2567,.F.);
#3894=ORIENTED_EDGE('',*,*,#2545,.F.);
#4040=CYLINDRICAL_SURFACE('',#4560,3.);
#4041=CYLINDRICAL_SURFACE('',#4579,0.5);
#4042=CYLINDRICAL_SURFACE('',#4581,3.5);
#4043=CYLINDRICAL_SURFACE('',#4582,24.7141941620437);
#4044=CYLINDRICAL_SURFACE('',#4583,9.);
#4045=CYLINDRICAL_SURFACE('',#4585,9.);
#4046=CYLINDRICAL_SURFACE('',#4586,4.445);
#4047=CYLINDRICAL_SURFACE('',#4588,4.445);
#4048=CYLINDRICAL_SURFACE('',#4592,3.99999999999999);
#4049=CYLINDRICAL_SURFACE('',#4596,4.00000000000001);
#4050=CYLINDRICAL_SURFACE('',#4600,4.00000000000001);
#4051=CYLINDRICAL_SURFACE('',#4604,4.00000000000001);
#4052=CYLINDRICAL_SURFACE('',#4607,6.99999999999999);
#4053=CYLINDRICAL_SURFACE('',#4610,9.9094315895918);
#4054=CYLINDRICAL_SURFACE('',#4613,5.);
#4055=CYLINDRICAL_SURFACE('',#4617,5.99999999999999);
#4056=CYLINDRICAL_SURFACE('',#4621,5.99999999999999);
#4057=CYLINDRICAL_SURFACE('',#4625,7.);
#4211=ADVANCED_FACE('',(#328),#4040,.T.);
#4212=ADVANCED_FACE('',(#329),#159,.T.);
#4213=ADVANCED_FACE('',(#330,#110),#160,.T.);
#4214=ADVANCED_FACE('',(#331),#161,.T.);
#4215=ADVANCED_FACE('',(#332,#111),#162,.T.);
#4216=ADVANCED_FACE('',(#333),#4041,.F.);
#4217=ADVANCED_FACE('',(#334),#4042,.T.);
#4218=ADVANCED_FACE('',(#335),#4043,.F.);
#4219=ADVANCED_FACE('',(#336),#4044,.T.);
#4220=ADVANCED_FACE('',(#337),#163,.T.);
#4221=ADVANCED_FACE('',(#338),#4045,.T.);
#4222=ADVANCED_FACE('',(#339),#4046,.F.);
#4223=ADVANCED_FACE('',(#340),#164,.T.);
#4224=ADVANCED_FACE('',(#341),#4047,.F.);
#4225=ADVANCED_FACE('',(#342),#165,.T.);
#4226=ADVANCED_FACE('',(#343),#4048,.F.);
#4227=ADVANCED_FACE('',(#344),#166,.T.);
#4228=ADVANCED_FACE('',(#345),#4049,.F.);
#4229=ADVANCED_FACE('',(#346),#167,.T.);
#4230=ADVANCED_FACE('',(#347),#4050,.F.);
#4231=ADVANCED_FACE('',(#348),#168,.T.);
#4232=ADVANCED_FACE('',(#349),#4051,.F.);
#4233=ADVANCED_FACE('',(#350),#4052,.T.);
#4234=ADVANCED_FACE('',(#351),#4053,.F.);
#4235=ADVANCED_FACE('',(#352),#4054,.F.);
#4236=ADVANCED_FACE('',(#353),#169,.T.);
#4237=ADVANCED_FACE('',(#354),#4055,.T.);
#4238=ADVANCED_FACE('',(#355),#170,.T.);
#4239=ADVANCED_FACE('',(#356),#4056,.T.);
#4240=ADVANCED_FACE('',(#357),#171,.T.);
#4241=ADVANCED_FACE('',(#358),#4057,.T.);
#4242=ADVANCED_FACE('',(#359),#172,.T.);
#4243=ADVANCED_FACE('',(#360,#112,#113),#173,.T.);
#4244=ADVANCED_FACE('',(#361,#114,#115),#174,.F.);
#4265=CLOSED_SHELL('',(#4211,#4212,#4213,#4214,#4215,#4216,#4217,#4218,
#4219,#4220,#4221,#4222,#4223,#4224,#4225,#4226,#4227,#4228,#4229,#4230,
#4231,#4232,#4233,#4234,#4235,#4236,#4237,#4238,#4239,#4240,#4241,#4242,
#4243,#4244));
#4559=AXIS2_PLACEMENT_3D('',#51251,#5236,#5237);
#4560=AXIS2_PLACEMENT_3D('',#51252,#5238,#5239);
#4561=AXIS2_PLACEMENT_3D('',#51255,#5240,#5241);
#4562=AXIS2_PLACEMENT_3D('',#51259,#5243,#5244);
#4563=AXIS2_PLACEMENT_3D('',#51263,#5246,#5247);
#4564=AXIS2_PLACEMENT_3D('',#51270,#5249,#5250);
#4565=AXIS2_PLACEMENT_3D('',#51274,#5252,#5253);
#4566=AXIS2_PLACEMENT_3D('',#51280,#5257,#5258);
#4567=AXIS2_PLACEMENT_3D('',#51284,#5260,#5261);
#4568=AXIS2_PLACEMENT_3D('',#51288,#5263,#5264);
#4569=AXIS2_PLACEMENT_3D('',#51290,#5265,#5266);
#4570=AXIS2_PLACEMENT_3D('',#51292,#5267,#5268);
#4571=AXIS2_PLACEMENT_3D('',#51297,#5271,#5272);
#4572=AXIS2_PLACEMENT_3D('',#51298,#5273,#5274);
#4573=AXIS2_PLACEMENT_3D('',#51302,#5277,#5278);
#4574=AXIS2_PLACEMENT_3D('',#51306,#5280,#5281);
#4575=AXIS2_PLACEMENT_3D('',#51308,#5282,#5283);
#4576=AXIS2_PLACEMENT_3D('',#51310,#5284,#5285);
#4577=AXIS2_PLACEMENT_3D('',#51313,#5287,#5288);
#4578=AXIS2_PLACEMENT_3D('',#51315,#5289,#5290);
#4579=AXIS2_PLACEMENT_3D('',#51316,#5291,#5292);
#4580=AXIS2_PLACEMENT_3D('',#51318,#5293,#5294);
#4581=AXIS2_PLACEMENT_3D('',#51320,#5296,#5297);
#4582=AXIS2_PLACEMENT_3D('',#51323,#5300,#5301);
#4583=AXIS2_PLACEMENT_3D('',#51325,#5303,#5304);
#4584=AXIS2_PLACEMENT_3D('',#51327,#5306,#5307);
#4585=AXIS2_PLACEMENT_3D('',#51329,#5309,#5310);
#4586=AXIS2_PLACEMENT_3D('',#51330,#5311,#5312);
#4587=AXIS2_PLACEMENT_3D('',#51332,#5314,#5315);
#4588=AXIS2_PLACEMENT_3D('',#51336,#5318,#5319);
#4589=AXIS2_PLACEMENT_3D('',#51338,#5320,#5321);
#4590=AXIS2_PLACEMENT_3D('',#51341,#5323,#5324);
#4591=AXIS2_PLACEMENT_3D('',#51342,#5325,#5326);
#4592=AXIS2_PLACEMENT_3D('',#51351,#5331,#5332);
#4593=AXIS2_PLACEMENT_3D('',#51353,#5333,#5334);
#4594=AXIS2_PLACEMENT_3D('',#51355,#5335,#5336);
#4595=AXIS2_PLACEMENT_3D('',#51357,#5338,#5339);
#4596=AXIS2_PLACEMENT_3D('',#51363,#5343,#5344);
#4597=AXIS2_PLACEMENT_3D('',#51365,#5345,#5346);
#4598=AXIS2_PLACEMENT_3D('',#51367,#5347,#5348);
#4599=AXIS2_PLACEMENT_3D('',#51369,#5350,#5351);
#4600=AXIS2_PLACEMENT_3D('',#51375,#5355,#5356);
#4601=AXIS2_PLACEMENT_3D('',#51377,#5357,#5358);
#4602=AXIS2_PLACEMENT_3D('',#51379,#5359,#5360);
#4603=AXIS2_PLACEMENT_3D('',#51381,#5362,#5363);
#4604=AXIS2_PLACEMENT_3D('',#51387,#5367,#5368);
#4605=AXIS2_PLACEMENT_3D('',#51388,#5369,#5370);
#4606=AXIS2_PLACEMENT_3D('',#51389,#5371,#5372);
#4607=AXIS2_PLACEMENT_3D('',#51390,#5373,#5374);
#4608=AXIS2_PLACEMENT_3D('',#51393,#5375,#5376);
#4609=AXIS2_PLACEMENT_3D('',#51397,#5378,#5379);
#4610=AXIS2_PLACEMENT_3D('',#51399,#5381,#5382);
#4611=AXIS2_PLACEMENT_3D('',#51400,#5383,#5384);
#4612=AXIS2_PLACEMENT_3D('',#51401,#5385,#5386);
#4613=AXIS2_PLACEMENT_3D('',#51402,#5387,#5388);
#4614=AXIS2_PLACEMENT_3D('',#51404,#5389,#5390);
#4615=AXIS2_PLACEMENT_3D('',#51406,#5391,#5392);
#4616=AXIS2_PLACEMENT_3D('',#51408,#5394,#5395);
#4617=AXIS2_PLACEMENT_3D('',#51414,#5399,#5400);
#4618=AXIS2_PLACEMENT_3D('',#51416,#5401,#5402);
#4619=AXIS2_PLACEMENT_3D('',#51418,#5403,#5404);
#4620=AXIS2_PLACEMENT_3D('',#51420,#5406,#5407);
#4621=AXIS2_PLACEMENT_3D('',#51426,#5411,#5412);
#4622=AXIS2_PLACEMENT_3D('',#51428,#5413,#5414);
#4623=AXIS2_PLACEMENT_3D('',#51430,#5415,#5416);
#4624=AXIS2_PLACEMENT_3D('',#51432,#5418,#5419);
#4625=AXIS2_PLACEMENT_3D('',#51438,#5423,#5424);
#4626=AXIS2_PLACEMENT_3D('',#51440,#5425,#5426);
#4627=AXIS2_PLACEMENT_3D('',#51442,#5427,#5428);
#4628=AXIS2_PLACEMENT_3D('',#51444,#5430,#5431);
#4629=AXIS2_PLACEMENT_3D('',#51447,#5434,#5435);
#4630=AXIS2_PLACEMENT_3D('',#51448,#5436,#5437);
#5236=DIRECTION('axis',(0.,0.,1.));
#5237=DIRECTION('refdir',(1.,0.,0.));
#5238=DIRECTION('center_axis',(1.,0.,0.));
#5239=DIRECTION('ref_axis',(0.,0.707106781186547,-0.707106781186548));
#5240=DIRECTION('center_axis',(1.,4.23704587765192E-32,0.));
#5241=DIRECTION('ref_axis',(-2.99604387228618E-32,0.707106781186547,-0.707106781186548));
#5242=DIRECTION('',(1.,0.,0.));
#5243=DIRECTION('center_axis',(-1.,-4.44089209850062E-15,0.));
#5244=DIRECTION('ref_axis',(-3.14018491736754E-15,0.707106781186547,-0.707106781186548));
#5245=DIRECTION('',(-1.,0.,0.));
#5246=DIRECTION('center_axis',(-1.,0.,0.));
#5247=DIRECTION('ref_axis',(0.,0.707106781186547,-0.707106781186548));
#5248=DIRECTION('',(-1.,0.,0.));
#5249=DIRECTION('center_axis',(1.,0.,0.));
#5250=DIRECTION('ref_axis',(0.,1.,0.));
#5251=DIRECTION('',(0.,0.,1.));
#5252=DIRECTION('center_axis',(1.,0.,0.));
#5253=DIRECTION('ref_axis',(0.,0.707106781186546,-0.707106781186549));
#5254=DIRECTION('',(0.,1.,0.));
#5255=DIRECTION('',(0.,0.,1.));
#5256=DIRECTION('',(0.,1.,0.));
#5257=DIRECTION('center_axis',(0.,-1.,0.));
#5258=DIRECTION('ref_axis',(1.,0.,0.));
#5259=DIRECTION('',(0.,0.,-1.));
#5260=DIRECTION('center_axis',(0.,1.,0.));
#5261=DIRECTION('ref_axis',(0.707106781186548,0.,0.707106781186548));
#5262=DIRECTION('',(1.,0.,0.));
#5263=DIRECTION('center_axis',(0.,1.,0.));
#5264=DIRECTION('ref_axis',(0.,0.,-1.));
#5265=DIRECTION('center_axis',(0.,1.,0.));
#5266=DIRECTION('ref_axis',(0.126759996397889,0.,-0.991933416774134));
#5267=DIRECTION('center_axis',(0.,1.,0.));
#5268=DIRECTION('ref_axis',(-0.785839144811216,0.,0.61843094883938));
#5269=DIRECTION('',(0.,0.,1.));
#5270=DIRECTION('',(-1.,0.,0.));
#5271=DIRECTION('center_axis',(0.,1.,0.));
#5272=DIRECTION('ref_axis',(1.,0.,0.));
#5273=DIRECTION('center_axis',(1.,4.44089209850062E-15,0.));
#5274=DIRECTION('ref_axis',(-4.44089209850062E-15,1.,0.));
#5275=DIRECTION('',(0.,0.,1.));
#5276=DIRECTION('',(-4.44089209850062E-15,1.,0.));
#5277=DIRECTION('center_axis',(0.,1.,0.));
#5278=DIRECTION('ref_axis',(-1.,0.,0.));
#5279=DIRECTION('',(0.,0.,-1.));
#5280=DIRECTION('center_axis',(0.,-1.,0.));
#5281=DIRECTION('ref_axis',(-0.785839144811216,0.,0.61843094883938));
#5282=DIRECTION('center_axis',(0.,-1.,0.));
#5283=DIRECTION('ref_axis',(0.126759996397889,0.,-0.991933416774134));
#5284=DIRECTION('center_axis',(0.,-1.,0.));
#5285=DIRECTION('ref_axis',(0.,0.,-1.));
#5286=DIRECTION('',(-1.,0.,0.));
#5287=DIRECTION('center_axis',(0.,-1.,0.));
#5288=DIRECTION('ref_axis',(0.707106781186548,0.,0.707106781186548));
#5289=DIRECTION('center_axis',(0.,-1.,0.));
#5290=DIRECTION('ref_axis',(1.,0.,0.));
#5291=DIRECTION('center_axis',(-1.,0.,0.));
#5292=DIRECTION('ref_axis',(0.,0.707106781186546,-0.707106781186549));
#5293=DIRECTION('center_axis',(-1.,-4.23704587765192E-32,0.));
#5294=DIRECTION('ref_axis',(-2.99604387228617E-32,0.707106781186546,-0.707106781186549));
#5295=DIRECTION('',(1.,0.,0.));
#5296=DIRECTION('center_axis',(0.,1.,0.));
#5297=DIRECTION('ref_axis',(-0.785839144811216,0.,0.61843094883938));
#5298=DIRECTION('',(4.23704587765192E-32,-1.,0.));
#5299=DIRECTION('',(0.,1.,0.));
#5300=DIRECTION('center_axis',(0.,1.,0.));
#5301=DIRECTION('ref_axis',(0.126759996397889,0.,-0.991933416774134));
#5302=DIRECTION('',(0.,-1.,0.));
#5303=DIRECTION('center_axis',(-4.44089209850062E-15,1.,0.));
#5304=DIRECTION('ref_axis',(0.707106781186548,3.14018491736755E-15,0.707106781186548));
#5305=DIRECTION('',(4.44089209850062E-15,-1.,0.));
#5306=DIRECTION('center_axis',(0.,0.,1.));
#5307=DIRECTION('ref_axis',(1.,0.,0.));
#5308=DIRECTION('',(0.,1.,0.));
#5309=DIRECTION('center_axis',(0.,-1.,0.));
#5310=DIRECTION('ref_axis',(0.,0.,-1.));
#5311=DIRECTION('center_axis',(0.,1.,0.));
#5312=DIRECTION('ref_axis',(1.,0.,0.));
#5313=DIRECTION('',(0.,1.,0.));
#5314=DIRECTION('center_axis',(-1.,-4.23704587765192E-32,0.));
#5315=DIRECTION('ref_axis',(4.23704587765192E-32,-1.,0.));
#5316=DIRECTION('',(0.,0.,1.));
#5317=DIRECTION('',(-4.23704587765192E-32,1.,0.));
#5318=DIRECTION('center_axis',(0.,0.,1.));
#5319=DIRECTION('ref_axis',(1.,0.,0.));
#5320=DIRECTION('center_axis',(0.,0.,-1.));
#5321=DIRECTION('ref_axis',(1.,0.,0.));
#5322=DIRECTION('',(0.,0.,1.));
#5323=DIRECTION('center_axis',(0.,0.,-1.));
#5324=DIRECTION('ref_axis',(1.,0.,0.));
#5325=DIRECTION('center_axis',(-1.,0.,0.));
#5326=DIRECTION('ref_axis',(0.,-1.,0.));
#5327=DIRECTION('',(0.,-1.,0.));
#5328=DIRECTION('',(0.,0.,1.));
#5329=DIRECTION('',(0.,-1.,0.));
#5330=DIRECTION('',(0.,0.,1.));
#5331=DIRECTION('center_axis',(0.,0.,1.));
#5332=DIRECTION('ref_axis',(1.,-2.7755575615629E-16,0.));
#5333=DIRECTION('center_axis',(0.,0.,-1.));
#5334=DIRECTION('ref_axis',(1.,-2.7755575615629E-16,0.));
#5335=DIRECTION('center_axis',(0.,0.,-1.));
#5336=DIRECTION('ref_axis',(1.,-2.7755575615629E-16,0.));
#5337=DIRECTION('',(0.,0.,1.));
#5338=DIRECTION('center_axis',(-1.29472072842584E-15,-1.,0.));
#5339=DIRECTION('ref_axis',(1.,-1.29472072842584E-15,0.));
#5340=DIRECTION('',(1.,-1.29472072842584E-15,0.));
#5341=DIRECTION('',(1.,-1.29472072842584E-15,0.));
#5342=DIRECTION('',(0.,0.,1.));
#5343=DIRECTION('center_axis',(0.,0.,1.));
#5344=DIRECTION('ref_axis',(0.,1.,0.));
#5345=DIRECTION('center_axis',(0.,0.,-1.));
#5346=DIRECTION('ref_axis',(0.,1.,0.));
#5347=DIRECTION('center_axis',(0.,0.,-1.));
#5348=DIRECTION('ref_axis',(0.,1.,0.));
#5349=DIRECTION('',(0.,0.,1.));
#5350=DIRECTION('center_axis',(1.,0.,0.));
#5351=DIRECTION('ref_axis',(0.,1.,0.));
#5352=DIRECTION('',(0.,1.,0.));
#5353=DIRECTION('',(0.,1.,0.));
#5354=DIRECTION('',(0.,0.,1.));
#5355=DIRECTION('center_axis',(0.,0.,1.));
#5356=DIRECTION('ref_axis',(-1.,-1.66533453693773E-15,0.));
#5357=DIRECTION('center_axis',(0.,0.,-1.));
#5358=DIRECTION('ref_axis',(-1.,-1.66533453693773E-15,0.));
#5359=DIRECTION('center_axis',(0.,0.,-1.));
#5360=DIRECTION('ref_axis',(-1.,-1.66533453693773E-15,0.));
#5361=DIRECTION('',(0.,0.,1.));
#5362=DIRECTION('center_axis',(-8.09200455266149E-16,1.,0.));
#5363=DIRECTION('ref_axis',(-1.,-8.09200455266149E-16,0.));
#5364=DIRECTION('',(-1.,-8.09200455266149E-16,0.));
#5365=DIRECTION('',(-1.,-8.09200455266149E-16,0.));
#5366=DIRECTION('',(0.,0.,1.));
#5367=DIRECTION('center_axis',(0.,0.,1.));
#5368=DIRECTION('ref_axis',(2.22044604925031E-15,-1.,0.));
#5369=DIRECTION('center_axis',(0.,0.,-1.));
#5370=DIRECTION('ref_axis',(2.22044604925031E-15,-1.,0.));
#5371=DIRECTION('center_axis',(0.,0.,-1.));
#5372=DIRECTION('ref_axis',(2.22044604925031E-15,-1.,0.));
#5373=DIRECTION('center_axis',(0.,0.,1.));
#5374=DIRECTION('ref_axis',(1.58603289232165E-16,1.,0.));
#5375=DIRECTION('center_axis',(0.,0.,1.));
#5376=DIRECTION('ref_axis',(1.58603289232165E-16,1.,0.));
#5377=DIRECTION('',(0.,0.,1.));
#5378=DIRECTION('center_axis',(0.,0.,1.));
#5379=DIRECTION('ref_axis',(1.58603289232165E-16,1.,0.));
#5380=DIRECTION('',(0.,0.,1.));
#5381=DIRECTION('center_axis',(0.,0.,1.));
#5382=DIRECTION('ref_axis',(0.559779357098146,-0.828641702647644,0.));
#5383=DIRECTION('center_axis',(0.,0.,1.));
#5384=DIRECTION('ref_axis',(0.559779357098146,-0.828641702647644,0.));
#5385=DIRECTION('center_axis',(0.,0.,-1.));
#5386=DIRECTION('ref_axis',(0.559779357098146,-0.828641702647644,0.));
#5387=DIRECTION('center_axis',(0.,0.,1.));
#5388=DIRECTION('ref_axis',(-1.,0.,0.));
#5389=DIRECTION('center_axis',(0.,0.,1.));
#5390=DIRECTION('ref_axis',(-1.,0.,0.));
#5391=DIRECTION('center_axis',(0.,0.,-1.));
#5392=DIRECTION('ref_axis',(-1.,0.,0.));
#5393=DIRECTION('',(0.,0.,1.));
#5394=DIRECTION('center_axis',(1.90049007730895E-14,-1.,0.));
#5395=DIRECTION('ref_axis',(1.,1.90049007730895E-14,0.));
#5396=DIRECTION('',(1.,1.90049007730895E-14,0.));
#5397=DIRECTION('',(1.,1.90049007730895E-14,0.));
#5398=DIRECTION('',(0.,0.,1.));
#5399=DIRECTION('center_axis',(0.,0.,1.));
#5400=DIRECTION('ref_axis',(1.,0.,0.));
#5401=DIRECTION('center_axis',(0.,0.,1.));
#5402=DIRECTION('ref_axis',(1.,0.,0.));
#5403=DIRECTION('center_axis',(0.,0.,1.));
#5404=DIRECTION('ref_axis',(1.,0.,0.));
#5405=DIRECTION('',(0.,0.,1.));
#5406=DIRECTION('center_axis',(1.,0.,0.));
#5407=DIRECTION('ref_axis',(0.,1.,0.));
#5408=DIRECTION('',(0.,1.,0.));
#5409=DIRECTION('',(0.,1.,0.));
#5410=DIRECTION('',(0.,0.,1.));
#5411=DIRECTION('center_axis',(0.,0.,1.));
#5412=DIRECTION('ref_axis',(-1.48029736616688E-15,-1.,0.));
#5413=DIRECTION('center_axis',(0.,0.,1.));
#5414=DIRECTION('ref_axis',(-1.48029736616688E-15,-1.,0.));
#5415=DIRECTION('center_axis',(0.,0.,1.));
#5416=DIRECTION('ref_axis',(-1.48029736616688E-15,-1.,0.));
#5417=DIRECTION('',(0.,0.,1.));
#5418=DIRECTION('center_axis',(0.,-1.,0.));
#5419=DIRECTION('ref_axis',(1.,0.,0.));
#5420=DIRECTION('',(1.,0.,0.));
#5421=DIRECTION('',(1.,0.,0.));
#5422=DIRECTION('',(0.,0.,1.));
#5423=DIRECTION('center_axis',(0.,0.,1.));
#5424=DIRECTION('ref_axis',(-1.,0.,0.));
#5425=DIRECTION('center_axis',(0.,0.,1.));
#5426=DIRECTION('ref_axis',(-1.,0.,0.));
#5427=DIRECTION('center_axis',(0.,0.,1.));
#5428=DIRECTION('ref_axis',(-1.,0.,0.));
#5429=DIRECTION('',(0.,0.,1.));
#5430=DIRECTION('center_axis',(-1.,-1.44006500428221E-15,0.));
#5431=DIRECTION('ref_axis',(1.44006500428221E-15,-1.,0.));
#5432=DIRECTION('',(1.44006500428221E-15,-1.,0.));
#5433=DIRECTION('',(1.44006500428221E-15,-1.,0.));
#5434=DIRECTION('center_axis',(0.,0.,1.));
#5435=DIRECTION('ref_axis',(1.,0.,0.));
#5436=DIRECTION('center_axis',(0.,0.,1.));
#5437=DIRECTION('ref_axis',(1.,0.,0.));
#51251=CARTESIAN_POINT('',(0.,0.,0.));
#51252=CARTESIAN_POINT('Origin',(376.324799934857,-11.9861373773513,-27.0570908269895));
#51253=CARTESIAN_POINT('',(339.771799934857,-10.9861373773513,-29.8855179517357));
#51254=CARTESIAN_POINT('',(339.771799934857,-8.98613737735134,-27.0570908269895));
#51255=CARTESIAN_POINT('Origin',(339.771799934857,-11.9861373773513,-27.0570908269895));
#51256=CARTESIAN_POINT('',(380.681799934857,-8.98613737735134,-27.0570908269895));
#51257=CARTESIAN_POINT('',(376.324799934857,-8.98613737735134,-27.0570908269895));
#51258=CARTESIAN_POINT('',(380.681799934857,-10.9861373773513,-29.8855179517357));
#51259=CARTESIAN_POINT('Origin',(380.681799934857,-11.9861373773513,-27.0570908269895));
#51260=CARTESIAN_POINT('',(380.681635380396,-10.9861373773513,-29.8855179517357));
#51261=CARTESIAN_POINT('',(376.324799934857,-10.9861373773513,-29.8855179517357));
#51262=CARTESIAN_POINT('',(380.681635380396,-11.9861373773513,-30.0570908269895));
#51263=CARTESIAN_POINT('Origin',(380.681635380396,-11.9861373773513,-27.0570908269895));
#51264=CARTESIAN_POINT('',(339.720861706803,-11.9861373773513,-30.0570908269895));
#51265=CARTESIAN_POINT('',(376.324799934857,-11.9861373773513,-30.0570908269895));
#51266=CARTESIAN_POINT('Ctrl Pts',(339.720861706803,-11.9861373773513,-30.0570908269895));
#51267=CARTESIAN_POINT('Ctrl Pts',(339.753951191729,-11.6599132580678,-30.0570908269895));
#51268=CARTESIAN_POINT('Ctrl Pts',(339.771447804716,-11.3135279162041,-30.0012679867952));
#51269=CARTESIAN_POINT('Ctrl Pts',(339.771447804716,-10.9861373773513,-29.8855179517357));
#51270=CARTESIAN_POINT('Origin',(380.681635380396,-15.0708658676184,-30.0570908269895));
#51271=CARTESIAN_POINT('',(380.681635380396,-10.9861373773513,-27.5570908269895));
#51272=CARTESIAN_POINT('',(380.681635380396,-10.9861373773513,-30.0570908269895));
#51273=CARTESIAN_POINT('',(380.681635380396,-11.4861373773513,-28.0570908269895));
#51274=CARTESIAN_POINT('Origin',(380.681635380396,-11.4861373773513,-27.5570908269895));
#51275=CARTESIAN_POINT('',(380.681635380396,-15.0708658676184,-28.0570908269895));
#51276=CARTESIAN_POINT('',(380.681635380396,-15.0708658676184,-28.0570908269895));
#51277=CARTESIAN_POINT('',(380.681635380396,-15.0708658676184,-30.0570908269895));
#51278=CARTESIAN_POINT('',(380.681635380396,-15.0708658676184,-30.0570908269895));
#51279=CARTESIAN_POINT('',(380.681635380396,-15.0708658676184,-30.0570908269895));
#51280=CARTESIAN_POINT('Origin',(330.604799934857,-10.9861373773513,-30.0570908269895));
#51281=CARTESIAN_POINT('',(380.681799934857,-10.9861373773513,0.820909173010471));
#51282=CARTESIAN_POINT('',(380.681799934857,-10.9861373773513,-30.0570908269895));
#51283=CARTESIAN_POINT('',(371.681799934857,-10.9861373773513,9.82090917301047));
#51284=CARTESIAN_POINT('Origin',(371.681799934857,-10.9861373773512,0.820909173010471));
#51285=CARTESIAN_POINT('',(370.321612719089,-10.9861373773513,9.82090917301047));
#51286=CARTESIAN_POINT('',(391.564799934857,-10.9861373773513,9.82090917301047));
#51287=CARTESIAN_POINT('',(361.330051062071,-10.9861373773513,1.21054870903725));
#51288=CARTESIAN_POINT('Origin',(370.321612719089,-10.9861373773513,0.820909173010471));
#51289=CARTESIAN_POINT('',(342.448997804234,-10.9861373773513,-21.7410591318785));
#51290=CARTESIAN_POINT('Origin',(336.6390287719,-10.9861373773513,2.28050728087887));
#51291=CARTESIAN_POINT('',(339.771799934857,-10.9861373773513,-25.1429698676036));
#51292=CARTESIAN_POINT('Origin',(343.271799934857,-10.9861373773513,-25.1429698676036));
#51293=CARTESIAN_POINT('',(339.771799934857,-10.9861373773513,-27.5570908269895));
#51294=CARTESIAN_POINT('',(339.771799934857,-10.9861373773513,-30.0570908269895));
#51295=CARTESIAN_POINT('',(345.844799934857,-10.9861373773513,-27.5570908269895));
#51296=CARTESIAN_POINT('',(366.389317853224,-10.9861373773513,0.));
#51297=CARTESIAN_POINT('Origin',(370.834317853224,-10.9861373773513,0.));
#51298=CARTESIAN_POINT('Origin',(380.681799934857,-10.9861373773514,-30.0570908269895));
#51299=CARTESIAN_POINT('',(380.681799934857,-8.98613737735134,0.820909173010471));
#51300=CARTESIAN_POINT('',(380.681799934857,-8.98613737735134,-30.0570908269895));
#51301=CARTESIAN_POINT('',(380.681799934857,-10.4861373773513,0.820909173010471));
#51302=CARTESIAN_POINT('Origin',(391.564799934857,-8.98613737735134,-30.0570908269895));
#51303=CARTESIAN_POINT('',(339.771799934857,-8.98613737735134,-25.1429698676036));
#51304=CARTESIAN_POINT('',(339.771799934857,-8.98613737735134,-30.0570908269895));
#51305=CARTESIAN_POINT('',(342.448997804234,-8.98613737735134,-21.7410591318785));
#51306=CARTESIAN_POINT('Origin',(343.271799934857,-8.98613737735134,-25.1429698676036));
#51307=CARTESIAN_POINT('',(361.330051062071,-8.98613737735134,1.21054870903725));
#51308=CARTESIAN_POINT('Origin',(336.6390287719,-8.98613737735134,2.28050728087887));
#51309=CARTESIAN_POINT('',(370.321612719089,-8.98613737735134,9.82090917301047));
#51310=CARTESIAN_POINT('Origin',(370.321612719089,-8.98613737735134,0.820909173010471));
#51311=CARTESIAN_POINT('',(371.681799934857,-8.98613737735134,9.82090917301047));
#51312=CARTESIAN_POINT('',(330.604799934857,-8.98613737735134,9.82090917301047));
#51313=CARTESIAN_POINT('Origin',(371.681799934857,-8.98613737735143,0.820909173010471));
#51314=CARTESIAN_POINT('',(366.389317853224,-8.98613737735134,0.));
#51315=CARTESIAN_POINT('Origin',(370.834317853224,-8.98613737735134,0.));
#51316=CARTESIAN_POINT('Origin',(345.844799934857,-11.4861373773513,-27.5570908269895));
#51317=CARTESIAN_POINT('',(339.771799934857,-11.4861373773513,-28.0570908269895));
#51318=CARTESIAN_POINT('Origin',(339.771799934857,-11.4861373773513,-27.5570908269895));
#51319=CARTESIAN_POINT('',(345.844799934857,-11.4861373773513,-28.0570908269895));
#51320=CARTESIAN_POINT('Origin',(343.271799934857,-10.9861373773513,-25.1429698676036));
#51321=CARTESIAN_POINT('',(339.771799934857,-10.9861373773513,-25.1429698676036));
#51322=CARTESIAN_POINT('',(342.448997804234,-10.9861373773513,-21.7410591318785));
#51323=CARTESIAN_POINT('Origin',(336.6390287719,-10.9861373773513,2.28050728087887));
#51324=CARTESIAN_POINT('',(361.330051062071,-10.9861373773513,1.21054870903726));
#51325=CARTESIAN_POINT('Origin',(371.681799934857,-10.4861373773514,0.820909173010471));
#51326=CARTESIAN_POINT('',(371.681799934857,-10.4861373773514,9.82090917301047));
#51327=CARTESIAN_POINT('Origin',(361.084799934857,-9.98613737735134,9.82090917301047));
#51328=CARTESIAN_POINT('',(370.321612719089,-10.9861373773513,9.82090917301047));
#51329=CARTESIAN_POINT('Origin',(370.321612719089,-10.9861373773513,0.820909173010471));
#51330=CARTESIAN_POINT('Origin',(370.834317853224,-10.9861373773513,0.));
#51331=CARTESIAN_POINT('',(366.389317853224,-10.9861373773513,5.44355502220999E-16));
#51332=CARTESIAN_POINT('Origin',(339.771799934857,-8.98613737735134,-30.0570908269895));
#51333=CARTESIAN_POINT('',(339.771799934857,-10.9861373773513,-28.0570908269895));
#51334=CARTESIAN_POINT('',(339.771799934857,-10.9861373773513,-30.0570908269895));
#51335=CARTESIAN_POINT('',(339.771799934857,-15.8361373773513,-28.0570908269895));
#51336=CARTESIAN_POINT('Origin',(339.301914228765,-26.9411392547891,-30.0570908269895));
#51337=CARTESIAN_POINT('',(334.856914228765,-26.9411392547891,-30.0570908269895));
#51338=CARTESIAN_POINT('Origin',(339.301914228765,-26.9411392547891,-30.0570908269895));
#51339=CARTESIAN_POINT('',(334.856914228765,-26.9411392547891,-28.0570908269895));
#51340=CARTESIAN_POINT('',(334.856914228765,-26.9411392547891,-30.0570908269895));
#51341=CARTESIAN_POINT('Origin',(339.301914228765,-26.9411392547891,-28.0570908269895));
#51342=CARTESIAN_POINT('Origin',(387.676491751218,-26.4627140227474,-30.0570908269895));
#51343=CARTESIAN_POINT('',(387.676491751218,-26.4627140227474,-30.0570908269895));
#51344=CARTESIAN_POINT('',(387.676491751218,-27.3527140227474,-30.0570908269895));
#51345=CARTESIAN_POINT('',(387.676491751218,-26.4627140227474,-30.0570908269895));
#51346=CARTESIAN_POINT('',(387.676491751218,-27.3527140227474,-28.0570908269895));
#51347=CARTESIAN_POINT('',(387.676491751218,-27.3527140227474,-30.0570908269895));
#51348=CARTESIAN_POINT('',(387.676491751218,-26.4627140227474,-28.0570908269895));
#51349=CARTESIAN_POINT('',(387.676491751218,-26.4627140227474,-28.0570908269895));
#51350=CARTESIAN_POINT('',(387.676491751218,-26.4627140227474,-30.0570908269895));
#51351=CARTESIAN_POINT('Origin',(383.676491751218,-26.4627140227474,-30.0570908269895));
#51352=CARTESIAN_POINT('',(383.676491751218,-22.4627140227474,-30.0570908269895));
#51353=CARTESIAN_POINT('Origin',(383.676491751218,-26.4627140227474,-30.0570908269895));
#51354=CARTESIAN_POINT('',(383.676491751218,-22.4627140227474,-28.0570908269895));
#51355=CARTESIAN_POINT('Origin',(383.676491751218,-26.4627140227474,-28.0570908269895));
#51356=CARTESIAN_POINT('',(383.676491751218,-22.4627140227474,-30.0570908269895));
#51357=CARTESIAN_POINT('Origin',(380.246491751218,-22.4627140227474,-30.0570908269895));
#51358=CARTESIAN_POINT('',(380.246491751218,-22.4627140227474,-30.0570908269895));
#51359=CARTESIAN_POINT('',(380.246491751218,-22.4627140227474,-30.0570908269895));
#51360=CARTESIAN_POINT('',(380.246491751218,-22.4627140227474,-28.0570908269895));
#51361=CARTESIAN_POINT('',(380.246491751218,-22.4627140227474,-28.0570908269895));
#51362=CARTESIAN_POINT('',(380.246491751218,-22.4627140227474,-30.0570908269895));
#51363=CARTESIAN_POINT('Origin',(380.246491751218,-26.4627140227474,-30.0570908269895));
#51364=CARTESIAN_POINT('',(376.246491751218,-26.4627140227474,-30.0570908269895));
#51365=CARTESIAN_POINT('Origin',(380.246491751218,-26.4627140227474,-30.0570908269895));
#51366=CARTESIAN_POINT('',(376.246491751218,-26.4627140227474,-28.0570908269895));
#51367=CARTESIAN_POINT('Origin',(380.246491751218,-26.4627140227474,-28.0570908269895));
#51368=CARTESIAN_POINT('',(376.246491751218,-26.4627140227474,-30.0570908269895));
#51369=CARTESIAN_POINT('Origin',(376.246491751218,-27.3527140227474,-30.0570908269895));
#51370=CARTESIAN_POINT('',(376.246491751218,-27.3527140227474,-30.0570908269895));
#51371=CARTESIAN_POINT('',(376.246491751218,-27.3527140227474,-30.0570908269895));
#51372=CARTESIAN_POINT('',(376.246491751218,-27.3527140227474,-28.0570908269895));
#51373=CARTESIAN_POINT('',(376.246491751218,-27.3527140227474,-28.0570908269895));
#51374=CARTESIAN_POINT('',(376.246491751218,-27.3527140227474,-30.0570908269895));
#51375=CARTESIAN_POINT('Origin',(380.246491751218,-27.3527140227474,-30.0570908269895));
#51376=CARTESIAN_POINT('',(380.246491751218,-31.3527140227474,-30.0570908269895));
#51377=CARTESIAN_POINT('Origin',(380.246491751218,-27.3527140227474,-30.0570908269895));
#51378=CARTESIAN_POINT('',(380.246491751218,-31.3527140227474,-28.0570908269895));
#51379=CARTESIAN_POINT('Origin',(380.246491751218,-27.3527140227474,-28.0570908269895));
#51380=CARTESIAN_POINT('',(380.246491751218,-31.3527140227474,-30.0570908269895));
#51381=CARTESIAN_POINT('Origin',(383.676491751218,-31.3527140227474,-30.0570908269895));
#51382=CARTESIAN_POINT('',(383.676491751218,-31.3527140227474,-30.0570908269895));
#51383=CARTESIAN_POINT('',(383.676491751218,-31.3527140227474,-30.0570908269895));
#51384=CARTESIAN_POINT('',(383.676491751218,-31.3527140227474,-28.0570908269895));
#51385=CARTESIAN_POINT('',(383.676491751218,-31.3527140227474,-28.0570908269895));
#51386=CARTESIAN_POINT('',(383.676491751218,-31.3527140227474,-30.0570908269895));
#51387=CARTESIAN_POINT('Origin',(383.676491751218,-27.3527140227474,-30.0570908269895));
#51388=CARTESIAN_POINT('Origin',(383.676491751218,-27.3527140227474,-30.0570908269895));
#51389=CARTESIAN_POINT('Origin',(383.676491751218,-27.3527140227474,-28.0570908269895));
#51390=CARTESIAN_POINT('Origin',(337.604799934857,-25.8442305588067,-30.0570908269895));
#51391=CARTESIAN_POINT('',(335.409111459553,-19.197505642021,-30.0570908269895));
#51392=CARTESIAN_POINT('',(330.604799934857,-25.8442305588067,-30.0570908269895));
#51393=CARTESIAN_POINT('Origin',(337.604799934857,-25.8442305588067,-30.0570908269895));
#51394=CARTESIAN_POINT('',(330.604799934857,-25.8442305588067,-28.0570908269895));
#51395=CARTESIAN_POINT('',(330.604799934857,-25.8442305588067,-30.0570908269895));
#51396=CARTESIAN_POINT('',(335.409111459553,-19.197505642021,-28.0570908269895));
#51397=CARTESIAN_POINT('Origin',(337.604799934857,-25.8442305588067,-28.0570908269895));
#51398=CARTESIAN_POINT('',(335.409111459553,-19.197505642021,-30.0570908269895));
#51399=CARTESIAN_POINT('Origin',(329.862016215124,-10.9861373773514,-30.0570908269895));
#51400=CARTESIAN_POINT('Origin',(329.862016215124,-10.9861373773514,-30.0570908269895));
#51401=CARTESIAN_POINT('Origin',(329.862016215124,-10.9861373773514,-28.0570908269895));
#51402=CARTESIAN_POINT('Origin',(385.681635380396,-15.0708658676184,-30.0570908269895));
#51403=CARTESIAN_POINT('',(385.681635380396,-20.0708658676184,-30.0570908269895));
#51404=CARTESIAN_POINT('Origin',(385.681635380396,-15.0708658676184,-30.0570908269895));
#51405=CARTESIAN_POINT('',(385.681635380396,-20.0708658676184,-28.0570908269895));
#51406=CARTESIAN_POINT('Origin',(385.681635380396,-15.0708658676184,-28.0570908269895));
#51407=CARTESIAN_POINT('',(385.681635380396,-20.0708658676184,-30.0570908269895));
#51408=CARTESIAN_POINT('Origin',(385.564799934857,-20.0708658676184,-30.0570908269895));
#51409=CARTESIAN_POINT('',(385.564799934857,-20.0708658676184,-30.0570908269895));
#51410=CARTESIAN_POINT('',(385.564799934857,-20.0708658676184,-30.0570908269895));
#51411=CARTESIAN_POINT('',(385.564799934857,-20.0708658676184,-28.0570908269895));
#51412=CARTESIAN_POINT('',(385.564799934857,-20.0708658676184,-28.0570908269895));
#51413=CARTESIAN_POINT('',(385.564799934857,-20.0708658676184,-30.0570908269895));
#51414=CARTESIAN_POINT('Origin',(385.564799934857,-26.0708658676183,-30.0570908269895));
#51415=CARTESIAN_POINT('',(391.564799934857,-26.0708658676183,-30.0570908269895));
#51416=CARTESIAN_POINT('Origin',(385.564799934857,-26.0708658676183,-30.0570908269895));
#51417=CARTESIAN_POINT('',(391.564799934857,-26.0708658676183,-28.0570908269895));
#51418=CARTESIAN_POINT('Origin',(385.564799934857,-26.0708658676183,-28.0570908269895));
#51419=CARTESIAN_POINT('',(391.564799934857,-26.0708658676183,-30.0570908269895));
#51420=CARTESIAN_POINT('Origin',(391.564799934857,-28.3861373773513,-30.0570908269895));
#51421=CARTESIAN_POINT('',(391.564799934857,-28.3861373773513,-30.0570908269895));
#51422=CARTESIAN_POINT('',(391.564799934857,-34.3861373773513,-30.0570908269895));
#51423=CARTESIAN_POINT('',(391.564799934857,-28.3861373773513,-28.0570908269895));
#51424=CARTESIAN_POINT('',(391.564799934857,-34.3861373773513,-28.0570908269895));
#51425=CARTESIAN_POINT('',(391.564799934857,-28.3861373773513,-30.0570908269895));
#51426=CARTESIAN_POINT('Origin',(385.564799934857,-28.3861373773514,-30.0570908269895));
#51427=CARTESIAN_POINT('',(385.564799934857,-34.3861373773513,-30.0570908269895));
#51428=CARTESIAN_POINT('Origin',(385.564799934857,-28.3861373773514,-30.0570908269895));
#51429=CARTESIAN_POINT('',(385.564799934857,-34.3861373773513,-28.0570908269895));
#51430=CARTESIAN_POINT('Origin',(385.564799934857,-28.3861373773514,-28.0570908269895));
#51431=CARTESIAN_POINT('',(385.564799934857,-34.3861373773513,-30.0570908269895));
#51432=CARTESIAN_POINT('Origin',(337.604799934857,-34.3861373773513,-30.0570908269895));
#51433=CARTESIAN_POINT('',(337.604799934857,-34.3861373773513,-30.0570908269895));
#51434=CARTESIAN_POINT('',(330.604799934857,-34.3861373773513,-30.0570908269895));
#51435=CARTESIAN_POINT('',(337.604799934857,-34.3861373773513,-28.0570908269895));
#51436=CARTESIAN_POINT('',(330.604799934857,-34.3861373773513,-28.0570908269895));
#51437=CARTESIAN_POINT('',(337.604799934857,-34.3861373773513,-30.0570908269895));
#51438=CARTESIAN_POINT('Origin',(337.604799934857,-27.3861373773513,-30.0570908269895));
#51439=CARTESIAN_POINT('',(330.604799934857,-27.3861373773513,-30.0570908269895));
#51440=CARTESIAN_POINT('Origin',(337.604799934857,-27.3861373773513,-30.0570908269895));
#51441=CARTESIAN_POINT('',(330.604799934857,-27.3861373773513,-28.0570908269895));
#51442=CARTESIAN_POINT('Origin',(337.604799934857,-27.3861373773513,-28.0570908269895));
#51443=CARTESIAN_POINT('',(330.604799934857,-27.3861373773513,-30.0570908269895));
#51444=CARTESIAN_POINT('Origin',(330.604799934857,-25.8442305588067,-30.0570908269895));
#51445=CARTESIAN_POINT('',(330.604799934857,-25.8442305588067,-30.0570908269895));
#51446=CARTESIAN_POINT('',(330.604799934857,-25.8442305588067,-28.0570908269895));
#51447=CARTESIAN_POINT('Origin',(361.084799934857,-22.6861373773513,-28.0570908269895));
#51448=CARTESIAN_POINT('Origin',(361.084799934857,-22.6861373773513,-30.0570908269895));
#51541=UNCERTAINTY_MEASURE_WITH_UNIT(LENGTH_MEASURE(0.01),#51554,
'DISTANCE_ACCURACY_VALUE',
'Maximum model space distance between geometric entities at asserted c
onnectivities');
#51543=UNCERTAINTY_MEASURE_WITH_UNIT(LENGTH_MEASURE(0.01),#51554,
'DISTANCE_ACCURACY_VALUE',
'Maximum model space distance between geometric entities at asserted c
onnectivities');
#51551=(
GEOMETRIC_REPRESENTATION_CONTEXT(3)
GLOBAL_UNCERTAINTY_ASSIGNED_CONTEXT((#51541))
GLOBAL_UNIT_ASSIGNED_CONTEXT((#51554,#51556,#51557))
REPRESENTATION_CONTEXT('','3D')
);
#51553=(
GEOMETRIC_REPRESENTATION_CONTEXT(3)
GLOBAL_UNCERTAINTY_ASSIGNED_CONTEXT((#51543))
GLOBAL_UNIT_ASSIGNED_CONTEXT((#51554,#51556,#51557))
REPRESENTATION_CONTEXT('','3D')
);
#51554=(
LENGTH_UNIT()
NAMED_UNIT(*)
SI_UNIT(.MILLI.,.METRE.)
);
#51556=(
NAMED_UNIT(*)
PLANE_ANGLE_UNIT()
SI_UNIT($,.RADIAN.)
);
#51557=(
NAMED_UNIT(*)
SI_UNIT($,.STERADIAN.)
SOLID_ANGLE_UNIT()
);
#51565=SHAPE_DEFINITION_REPRESENTATION(#51574,#51591);
#51574=PRODUCT_DEFINITION_SHAPE('',$,#51601);
#51591=SHAPE_REPRESENTATION('',(#4559),#51551);
#51593=PRODUCT_DEFINITION_CONTEXT('part definition',#51622,'design');
#51601=PRODUCT_DEFINITION('Clamp_02','Clamp_02',#51610,#51593);
#51610=PRODUCT_DEFINITION_FORMATION('',$,#51631);
#51622=APPLICATION_CONTEXT(
'Core Data for Automotive Mechanical Design Process');
#51623=PRODUCT_CONTEXT('part definition',#51622,'mechanical');
#51631=PRODUCT('Clamp_02','Clamp_02',$,(#51623));
#51634=PRESENTATION_STYLE_ASSIGNMENT((#51637));
#51637=SURFACE_STYLE_USAGE(.BOTH.,#51640);
#51640=SURFACE_SIDE_STYLE('',(#51643));
#51643=SURFACE_STYLE_FILL_AREA(#51646);
#51646=FILL_AREA_STYLE('Opaque(203,203,203)',(#51649));
#51649=FILL_AREA_STYLE_COLOUR('Opaque(203,203,203)',#51652);
#51652=COLOUR_RGB('Opaque(203,203,203)', 0.09019608, 0.27058824, 0.51372549);
ENDSEC;
END-ISO-10303-21;
